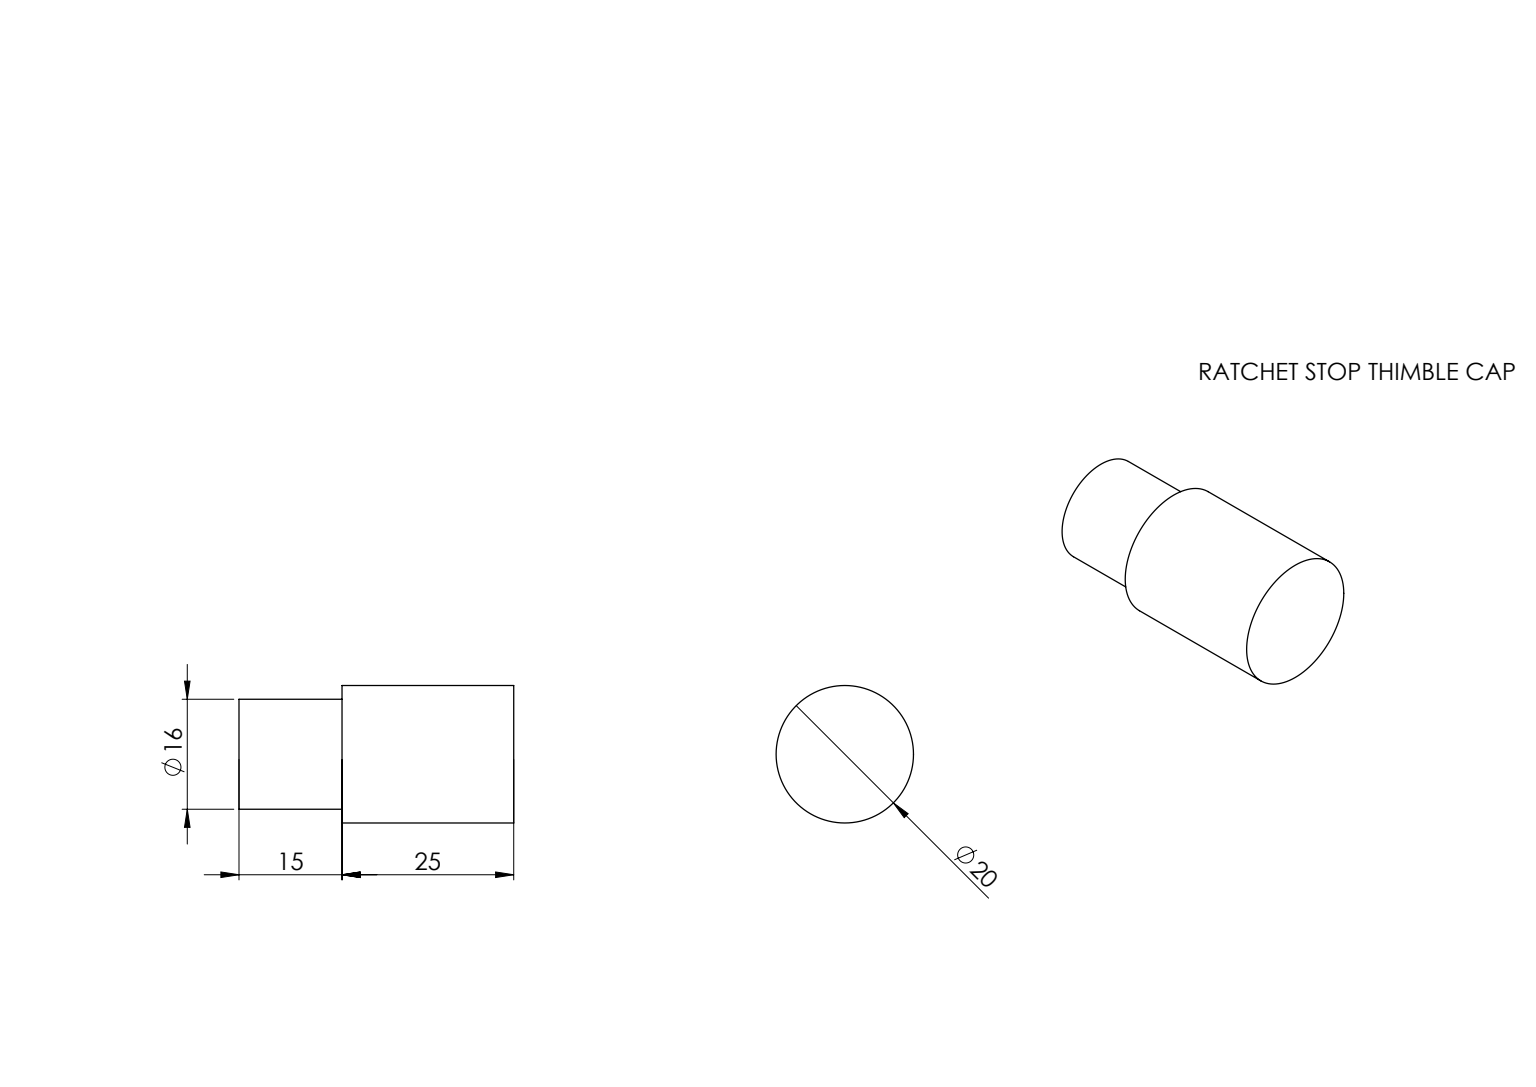
ISO-10303-21;
HEADER;
FILE_DESCRIPTION (('STEP AP214'),
    '1' );
FILE_NAME ('Ratchet Stop Thimble Cap.step',
    '2026-10-22T12:35:56',
    ( '' ),
    ( '' ),
    'SwSTEP 2.0',
    'SolidWorks 2026',
    '' );
FILE_SCHEMA (( 'AUTOMOTIVE_DESIGN' ));
ENDSEC;

DATA;
#21=PRESENTATION_STYLE_ASSIGNMENT (( #2824 ) ) ;
#28=EDGE_CURVE ( 'NONE', #1232, #2394, #2025, .T. ) ;
#41=CARTESIAN_POINT ( 'NONE',  ( 155.0000000000000284, -6.316519372592878167E-15, 2.499999999999999556 ) ) ;
#44=EDGE_CURVE ( 'NONE', #1232, #2037, #954, .T. ) ;
#58=VECTOR ( 'NONE', #2842, 1000.000000000000000 ) ;
#61=CLOSED_SHELL ( 'NONE', ( #1282, #587, #178, #1971, #3042, #967, #2402, #1991, #3073, #2520 ) ) ;
#68=CARTESIAN_POINT ( 'NONE',  ( 180.0000000000000284, -6.928842772166554697E-15, 7.500000000000000000 ) ) ;
#78=CARTESIAN_POINT ( 'NONE',  ( 180.0000000000000284, -6.928842772166554697E-15, 7.500000000000000000 ) ) ;
#80=DIRECTION ( 'NONE',  ( 1.000000000000000000, 0.000000000000000000, 0.000000000000000000 ) ) ;
#90=DIRECTION ( 'NONE',  ( -1.000000000000000000, -0.000000000000000000, -0.000000000000000000 ) ) ;
#91=VERTEX_POINT ( 'NONE', #398 ) ;
#94=SHAPE_DEFINITION_REPRESENTATION ( #2508, #2591 ) ;
#130=FACE_OUTER_BOUND ( 'NONE', #879, .T. ) ;
#132=CARTESIAN_POINT ( 'NONE',  ( 155.0000000000000284, -5.949125332848671934E-15, -0.5000000000000004441 ) ) ;
#142=ORIENTED_EDGE ( 'NONE', *, *, #1580, .F. ) ;
#150=CARTESIAN_POINT ( 'NONE',  ( 140.0000000000000000, -6.928842772166554697E-15, 15.50000000000000000 ) ) ;
#166=CARTESIAN_POINT ( 'NONE',  ( 140.0000000000000000, -6.928842772166554697E-15, 7.500000000000000000 ) ) ;
#178=ADVANCED_FACE ( 'NONE', ( #1464 ), #509, .T. ) ;
#189=( LENGTH_UNIT ( ) NAMED_UNIT ( * ) SI_UNIT ( .MILLI., .METRE. ) );
#194=CARTESIAN_POINT ( 'NONE',  ( 155.0000000000000284, -6.928842772166554697E-15, 7.500000000000000000 ) ) ;
#195=CIRCLE ( 'NONE', #1445, 10.00000000000000178 ) ;
#208=DIRECTION ( 'NONE',  ( 0.000000000000000000, 0.000000000000000000, 1.000000000000000000 ) ) ;
#212=CARTESIAN_POINT ( 'NONE',  ( 180.0000000000000284, -5.704195973019200848E-15, -2.500000000000002220 ) ) ;
#228=DIRECTION ( 'NONE',  ( 1.000000000000000000, 0.000000000000000000, 0.000000000000000000 ) ) ;
#245=ORIENTED_EDGE ( 'NONE', *, *, #981, .F. ) ;
#252=EDGE_CURVE ( 'NONE', #466, #91, #1941, .T. ) ;
#263=AXIS2_PLACEMENT_3D ( 'NONE', #1782, #798, #1552 ) ;
#286=CARTESIAN_POINT ( 'NONE',  ( 140.0000000000000000, -6.316519372592878167E-15, 2.499999999999999556 ) ) ;
#290=PRODUCT_DEFINITION_CONTEXT ( 'detailed design', #3029, 'design' ) ;
#298=EDGE_CURVE ( 'NONE', #3130, #2427, #2917, .T. ) ;
#304=CARTESIAN_POINT ( 'NONE',  ( 180.0000000000000284, -6.928842772166554697E-15, 7.500000000000000000 ) ) ;
#309=( NAMED_UNIT ( * ) SI_UNIT ( $, .STERADIAN. ) SOLID_ANGLE_UNIT ( ) );
#332=ORIENTED_EDGE ( 'NONE', *, *, #28, .F. ) ;
#338=FACE_OUTER_BOUND ( 'NONE', #1623, .T. ) ;
#339=AXIS2_PLACEMENT_3D ( 'NONE', #2130, #2093, #2543 ) ;
#347=CARTESIAN_POINT ( 'NONE',  ( 180.0000000000000284, -6.928842772166554697E-15, 17.50000000000000000 ) ) ;
#368=CARTESIAN_POINT ( 'NONE',  ( 140.0000000000000000, -6.928842772166554697E-15, 7.500000000000000000 ) ) ;
#395=AXIS2_PLACEMENT_3D ( 'NONE', #2044, #2788, #565 ) ;
#396=MECHANICAL_DESIGN_GEOMETRIC_PRESENTATION_REPRESENTATION('',(#2111),#1957);
#398=CARTESIAN_POINT ( 'NONE',  ( 155.0000000000000284, -6.928842772166554697E-15, 17.50000000000000000 ) ) ;
#407=DIRECTION ( 'NONE',  ( 0.000000000000000000, 0.000000000000000000, -1.000000000000000000 ) ) ;
#412=ORIENTED_EDGE ( 'NONE', *, *, #843, .T. ) ;
#418=PLANE ( 'NONE',  #2778 ) ;
#430=ORIENTED_EDGE ( 'NONE', *, *, #981, .T. ) ;
#433=DIRECTION ( 'NONE',  ( 1.000000000000000000, 0.000000000000000000, 0.000000000000000000 ) ) ;
#466=VERTEX_POINT ( 'NONE', #347 ) ;
#473=AXIS2_PLACEMENT_3D ( 'NONE', #1752, #228, #2224 ) ;
#479=VERTEX_POINT ( 'NONE', #286 ) ;
#498=ORIENTED_EDGE ( 'NONE', *, *, #1931, .T. ) ;
#509=CYLINDRICAL_SURFACE ( 'NONE', #747, 8.000000000000000000 ) ;
#554=DIRECTION ( 'NONE',  ( -1.000000000000000000, -0.000000000000000000, -0.000000000000000000 ) ) ;
#557=( LENGTH_UNIT ( ) NAMED_UNIT ( * ) SI_UNIT ( .MILLI., .METRE. ) );
#565=DIRECTION ( 'NONE',  ( 0.000000000000000000, 0.000000000000000000, 1.000000000000000000 ) ) ;
#583=CYLINDRICAL_SURFACE ( 'NONE', #2281, 10.00000000000000178 ) ;
#584=( NAMED_UNIT ( * ) PLANE_ANGLE_UNIT ( ) SI_UNIT ( $, .RADIAN. ) );
#587=ADVANCED_FACE ( 'NONE', ( #1804 ), #785, .F. ) ;
#597=CARTESIAN_POINT ( 'NONE',  ( 155.0000000000000284, -5.704195973019200848E-15, -2.500000000000002220 ) ) ;
#617=ORIENTED_EDGE ( 'NONE', *, *, #252, .T. ) ;
#633=( GEOMETRIC_REPRESENTATION_CONTEXT ( 3 ) GLOBAL_UNCERTAINTY_ASSIGNED_CONTEXT ( ( #2364 ) ) GLOBAL_UNIT_ASSIGNED_CONTEXT ( ( #189, #684, #1683 ) ) REPRESENTATION_CONTEXT ( 'NONE', 'WORKASPACE' ) );
#643=ORIENTED_EDGE ( 'NONE', *, *, #44, .T. ) ;
#644=DIRECTION ( 'NONE',  ( 0.000000000000000000, 0.000000000000000000, -1.000000000000000000 ) ) ;
#646=PLANE ( 'NONE',  #339 ) ;
#653=FACE_OUTER_BOUND ( 'NONE', #990, .T. ) ;
#663=ORIENTED_EDGE ( 'NONE', *, *, #843, .F. ) ;
#666=CARTESIAN_POINT ( 'NONE',  ( 155.0000000000000284, -6.928842772166554697E-15, 7.500000000000000000 ) ) ;
#672=CARTESIAN_POINT ( 'NONE',  ( 155.0000000000000284, -6.928842772166554697E-15, 7.500000000000000000 ) ) ;
#675=ORIENTED_EDGE ( 'NONE', *, *, #1886, .F. ) ;
#684=( NAMED_UNIT ( * ) PLANE_ANGLE_UNIT ( ) SI_UNIT ( $, .RADIAN. ) );
#712=DIRECTION ( 'NONE',  ( 1.000000000000000000, 0.000000000000000000, 0.000000000000000000 ) ) ;
#737=ORIENTED_EDGE ( 'NONE', *, *, #1525, .T. ) ;
#747=AXIS2_PLACEMENT_3D ( 'NONE', #194, #1501, #208 ) ;
#785=CYLINDRICAL_SURFACE ( 'NONE', #395, 5.000000000000000888 ) ;
#794=ORIENTED_EDGE ( 'NONE', *, *, #28, .T. ) ;
#798=DIRECTION ( 'NONE',  ( 1.000000000000000000, 0.000000000000000000, 0.000000000000000000 ) ) ;
#800=CARTESIAN_POINT ( 'NONE',  ( 155.0000000000000284, -6.928842772166554697E-15, 12.50000000000000000 ) ) ;
#843=EDGE_CURVE ( 'NONE', #2350, #2807, #1836, .T. ) ;
#863=CARTESIAN_POINT ( 'NONE',  ( 140.0000000000000000, -6.928842772166554697E-15, 12.50000000000000000 ) ) ;
#865=DIRECTION ( 'NONE',  ( 0.000000000000000000, 0.000000000000000000, 1.000000000000000000 ) ) ;
#873=UNCERTAINTY_MEASURE_WITH_UNIT (LENGTH_MEASURE( 1.000000000000000082E-05 ), #3007, 'distance_accuracy_value', 'NONE');
#878=CARTESIAN_POINT ( 'NONE',  ( 155.0000000000000284, -6.928842772166554697E-15, 7.500000000000000000 ) ) ;
#879=EDGE_LOOP ( 'NONE', ( #2061, #2408 ) ) ;
#903=PRODUCT_CONTEXT ( 'NONE', #969, 'mechanical' ) ;
#940=CARTESIAN_POINT ( 'NONE',  ( 180.0000000000000284, -5.704195973019200848E-15, -2.500000000000002220 ) ) ;
#954=CIRCLE ( 'NONE', #1215, 5.000000000000000000 ) ;
#955=DIRECTION ( 'NONE',  ( -1.000000000000000000, -0.000000000000000000, -0.000000000000000000 ) ) ;
#958=CARTESIAN_POINT ( 'NONE',  ( 180.0000000000000284, -6.928842772166554697E-15, 17.50000000000000000 ) ) ;
#963=FACE_OUTER_BOUND ( 'NONE', #1238, .T. ) ;
#967=ADVANCED_FACE ( 'NONE', ( #2453 ), #2960, .F. ) ;
#969=APPLICATION_CONTEXT ( 'automotive_design' ) ;
#981=EDGE_CURVE ( 'NONE', #2037, #479, #1478, .T. ) ;
#985=AXIS2_PLACEMENT_3D ( 'NONE', #1976, #2688, #2443 ) ;
#990=EDGE_LOOP ( 'NONE', ( #2913, #1504 ) ) ;
#1000=AXIS2_PLACEMENT_3D ( 'NONE', #672, #1412, #2437 ) ;
#1003=VECTOR ( 'NONE', #1553, 1000.000000000000000 ) ;
#1006=EDGE_CURVE ( 'NONE', #2037, #1232, #2098, .T. ) ;
#1017=( NAMED_UNIT ( * ) SI_UNIT ( $, .STERADIAN. ) SOLID_ANGLE_UNIT ( ) );
#1095=ORIENTED_EDGE ( 'NONE', *, *, #2970, .F. ) ;
#1111=CIRCLE ( 'NONE', #1320, 10.00000000000000178 ) ;
#1129=DIRECTION ( 'NONE',  ( 1.000000000000000000, 0.000000000000000000, 0.000000000000000000 ) ) ;
#1139=ADVANCED_BREP_SHAPE_REPRESENTATION ( '', ( #2105, #2878 ), #1375 ) ;
#1152=EDGE_LOOP ( 'NONE', ( #2145, #412, #1160, #2143 ) ) ;
#1160=ORIENTED_EDGE ( 'NONE', *, *, #2742, .T. ) ;
#1161=AXIS2_PLACEMENT_3D ( 'NONE', #1671, #2404, #2221 ) ;
#1207=ORIENTED_EDGE ( 'NONE', *, *, #2422, .T. ) ;
#1215=AXIS2_PLACEMENT_3D ( 'NONE', #1827, #1332, #1802 ) ;
#1219=CIRCLE ( 'NONE', #2885, 8.000000000000000000 ) ;
#1232=VERTEX_POINT ( 'NONE', #2371 ) ;
#1238=EDGE_LOOP ( 'NONE', ( #1589, #1095 ) ) ;
#1264=PRODUCT_DEFINITION ( 'UNKNOWN', '', #1910, #290 ) ;
#1265=AXIS2_PLACEMENT_3D ( 'NONE', #368, #80, #3066 ) ;
#1270=AXIS2_PLACEMENT_3D ( 'NONE', #78, #1129, #644 ) ;
#1282=ADVANCED_FACE ( 'NONE', ( #2116 ), #583, .T. ) ;
#1284=CARTESIAN_POINT ( 'NONE',  ( 140.0000000000000000, -6.928842772166554697E-15, 7.500000000000000000 ) ) ;
#1299=DIRECTION ( 'NONE',  ( 1.000000000000000000, 0.000000000000000000, 0.000000000000000000 ) ) ;
#1300=CIRCLE ( 'NONE', #263, 8.000000000000000000 ) ;
#1319=ORIENTED_EDGE ( 'NONE', *, *, #298, .F. ) ;
#1320=AXIS2_PLACEMENT_3D ( 'NONE', #878, #2334, #1388 ) ;
#1323=DIRECTION ( 'NONE',  ( 0.000000000000000000, 0.000000000000000000, 1.000000000000000000 ) ) ;
#1332=DIRECTION ( 'NONE',  ( 1.000000000000000000, 0.000000000000000000, 0.000000000000000000 ) ) ;
#1337=VECTOR ( 'NONE', #554, 1000.000000000000000 ) ;
#1342=VERTEX_POINT ( 'NONE', #150 ) ;
#1352=ORIENTED_EDGE ( 'NONE', *, *, #44, .F. ) ;
#1375=( GEOMETRIC_REPRESENTATION_CONTEXT ( 3 ) GLOBAL_UNCERTAINTY_ASSIGNED_CONTEXT ( ( #1894 ) ) GLOBAL_UNIT_ASSIGNED_CONTEXT ( ( #557, #584, #1017 ) ) REPRESENTATION_CONTEXT ( 'NONE', 'WORKASPACE' ) );
#1388=DIRECTION ( 'NONE',  ( 0.000000000000000000, 0.000000000000000000, -1.000000000000000000 ) ) ;
#1412=DIRECTION ( 'NONE',  ( -1.000000000000000000, -0.000000000000000000, -0.000000000000000000 ) ) ;
#1419=EDGE_LOOP ( 'NONE', ( #142, #1925, #1642, #1594 ) ) ;
#1431=CARTESIAN_POINT ( 'NONE',  ( 155.0000000000000284, -6.316519372592878167E-15, 2.499999999999999556 ) ) ;
#1445=AXIS2_PLACEMENT_3D ( 'NONE', #304, #2774, #2511 ) ;
#1454=FACE_BOUND ( 'NONE', #2335, .T. ) ;
#1459=AXIS2_PLACEMENT_3D ( 'NONE', #1800, #2389, #1891 ) ;
#1464=FACE_OUTER_BOUND ( 'NONE', #1152, .T. ) ;
#1472=CARTESIAN_POINT ( 'NONE',  ( 155.0000000000000284, -6.928842772166554697E-15, 15.50000000000000000 ) ) ;
#1478=LINE ( 'NONE', #1431, #3191 ) ;
#1492=CARTESIAN_POINT ( 'NONE',  ( 140.0000000000000000, -5.949125332848671934E-15, -0.5000000000000004441 ) ) ;
#1501=DIRECTION ( 'NONE',  ( -1.000000000000000000, -0.000000000000000000, -0.000000000000000000 ) ) ;
#1504=ORIENTED_EDGE ( 'NONE', *, *, #2742, .F. ) ;
#1525=EDGE_CURVE ( 'NONE', #1604, #1342, #2031, .T. ) ;
#1527=SURFACE_SIDE_STYLE ('',( #1547 ) ) ;
#1547=SURFACE_STYLE_FILL_AREA ( #2279 ) ;
#1552=DIRECTION ( 'NONE',  ( 0.000000000000000000, 0.000000000000000000, -1.000000000000000000 ) ) ;
#1553=DIRECTION ( 'NONE',  ( -1.000000000000000000, -0.000000000000000000, -0.000000000000000000 ) ) ;
#1571=CIRCLE ( 'NONE', #2302, 10.00000000000000178 ) ;
#1580=EDGE_CURVE ( 'NONE', #3130, #466, #195, .T. ) ;
#1589=ORIENTED_EDGE ( 'NONE', *, *, #1869, .F. ) ;
#1594=ORIENTED_EDGE ( 'NONE', *, *, #252, .F. ) ;
#1604=VERTEX_POINT ( 'NONE', #1472 ) ;
#1617=ORIENTED_EDGE ( 'NONE', *, *, #2613, .T. ) ;
#1618=CIRCLE ( 'NONE', #985, 8.000000000000000000 ) ;
#1622=CYLINDRICAL_SURFACE ( 'NONE', #2464, 8.000000000000000000 ) ;
#1623=EDGE_LOOP ( 'NONE', ( #1352, #1652 ) ) ;
#1637=ORIENTED_EDGE ( 'NONE', *, *, #2639, .F. ) ;
#1642=ORIENTED_EDGE ( 'NONE', *, *, #2970, .T. ) ;
#1648=DIRECTION ( 'NONE',  ( 1.000000000000000000, 0.000000000000000000, 0.000000000000000000 ) ) ;
#1652=ORIENTED_EDGE ( 'NONE', *, *, #1006, .F. ) ;
#1671=CARTESIAN_POINT ( 'NONE',  ( 155.0000000000000284, -6.928842772166554697E-15, 7.500000000000000000 ) ) ;
#1683=( NAMED_UNIT ( * ) SI_UNIT ( $, .STERADIAN. ) SOLID_ANGLE_UNIT ( ) );
#1696=CARTESIAN_POINT ( 'NONE',  ( 140.0000000000000000, -6.928842772166554697E-15, 7.500000000000000000 ) ) ;
#1711=EDGE_LOOP ( 'NONE', ( #643, #430, #2950, #332 ) ) ;
#1748=VECTOR ( 'NONE', #1750, 1000.000000000000000 ) ;
#1749=EDGE_LOOP ( 'NONE', ( #663, #675, #737, #1763 ) ) ;
#1750=DIRECTION ( 'NONE',  ( -1.000000000000000000, -0.000000000000000000, -0.000000000000000000 ) ) ;
#1752=CARTESIAN_POINT ( 'NONE',  ( 155.0000000000000284, -6.928842772166554697E-15, 7.500000000000000000 ) ) ;
#1763=ORIENTED_EDGE ( 'NONE', *, *, #2556, .T. ) ;
#1782=CARTESIAN_POINT ( 'NONE',  ( 155.0000000000000284, -6.928842772166554697E-15, 7.500000000000000000 ) ) ;
#1800=CARTESIAN_POINT ( 'NONE',  ( 180.0000000000000284, -6.928842772166554697E-15, 7.500000000000000000 ) ) ;
#1802=DIRECTION ( 'NONE',  ( 0.000000000000000000, 0.000000000000000000, -1.000000000000000000 ) ) ;
#1804=FACE_OUTER_BOUND ( 'NONE', #1711, .T. ) ;
#1827=CARTESIAN_POINT ( 'NONE',  ( 155.0000000000000284, -6.928842772166554697E-15, 7.500000000000000000 ) ) ;
#1831=FACE_OUTER_BOUND ( 'NONE', #1749, .T. ) ;
#1836=LINE ( 'NONE', #2100, #58 ) ;
#1837=DIRECTION ( 'NONE',  ( 1.000000000000000000, 0.000000000000000000, 0.000000000000000000 ) ) ;
#1869=EDGE_CURVE ( 'NONE', #91, #2427, #1878, .T. ) ;
#1878=CIRCLE ( 'NONE', #473, 10.00000000000000178 ) ;
#1886=EDGE_CURVE ( 'NONE', #1604, #2350, #1618, .T. ) ;
#1891=DIRECTION ( 'NONE',  ( 0.000000000000000000, 0.000000000000000000, 1.000000000000000000 ) ) ;
#1894=UNCERTAINTY_MEASURE_WITH_UNIT (LENGTH_MEASURE( 1.000000000000000082E-05 ), #557, 'distance_accuracy_value', 'NONE');
#1910=PRODUCT_DEFINITION_FORMATION_WITH_SPECIFIED_SOURCE ( 'ANY', '', #2771, .NOT_KNOWN. ) ;
#1919=DIRECTION ( 'NONE',  ( 0.000000000000000000, 0.000000000000000000, -1.000000000000000000 ) ) ;
#1925=ORIENTED_EDGE ( 'NONE', *, *, #298, .T. ) ;
#1931=EDGE_CURVE ( 'NONE', #2350, #1604, #1300, .T. ) ;
#1935=DIRECTION ( 'NONE',  ( 0.000000000000000000, 0.000000000000000000, -1.000000000000000000 ) ) ;
#1941=LINE ( 'NONE', #958, #1951 ) ;
#1951=VECTOR ( 'NONE', #2702, 1000.000000000000000 ) ;
#1957=( GEOMETRIC_REPRESENTATION_CONTEXT ( 3 ) GLOBAL_UNCERTAINTY_ASSIGNED_CONTEXT ( ( #873 ) ) GLOBAL_UNIT_ASSIGNED_CONTEXT ( ( #3007, #3022, #309 ) ) REPRESENTATION_CONTEXT ( 'NONE', 'WORKASPACE' ) );
#1965=DIRECTION ( 'NONE',  ( 1.000000000000000000, 0.000000000000000000, 0.000000000000000000 ) ) ;
#1971=ADVANCED_FACE ( 'NONE', ( #653, #2135 ), #3028, .F. ) ;
#1976=CARTESIAN_POINT ( 'NONE',  ( 155.0000000000000284, -6.928842772166554697E-15, 7.500000000000000000 ) ) ;
#1991=ADVANCED_FACE ( 'NONE', ( #2592 ), #2120, .T. ) ;
#2011=ORIENTED_EDGE ( 'NONE', *, *, #2422, .F. ) ;
#2025=LINE ( 'NONE', #800, #1003 ) ;
#2031=LINE ( 'NONE', #2480, #1337 ) ;
#2037=VERTEX_POINT ( 'NONE', #41 ) ;
#2042=AXIS2_PLACEMENT_3D ( 'NONE', #166, #2182, #2956 ) ;
#2044=CARTESIAN_POINT ( 'NONE',  ( 155.0000000000000284, -6.928842772166554697E-15, 7.500000000000000000 ) ) ;
#2061=ORIENTED_EDGE ( 'NONE', *, *, #2639, .T. ) ;
#2093=DIRECTION ( 'NONE',  ( 1.000000000000000000, 0.000000000000000000, 0.000000000000000000 ) ) ;
#2098=CIRCLE ( 'NONE', #1161, 5.000000000000000000 ) ;
#2100=CARTESIAN_POINT ( 'NONE',  ( 155.0000000000000284, -5.949125332848671934E-15, -0.5000000000000004441 ) ) ;
#2105=MANIFOLD_SOLID_BREP ( 'Boss-Extrude1', #61 ) ;
#2111=STYLED_ITEM ( 'NONE', ( #21 ), #1139 ) ;
#2116=FACE_OUTER_BOUND ( 'NONE', #1419, .T. ) ;
#2120=CYLINDRICAL_SURFACE ( 'NONE', #1459, 10.00000000000000178 ) ;
#2130=CARTESIAN_POINT ( 'NONE',  ( 155.0000000000000284, -6.928842772166554697E-15, 7.500000000000000000 ) ) ;
#2135=FACE_BOUND ( 'NONE', #2178, .T. ) ;
#2143=ORIENTED_EDGE ( 'NONE', *, *, #1525, .F. ) ;
#2145=ORIENTED_EDGE ( 'NONE', *, *, #1931, .F. ) ;
#2150=AXIS2_PLACEMENT_3D ( 'NONE', #2627, #1648, #1919 ) ;
#2178=EDGE_LOOP ( 'NONE', ( #1617, #1207 ) ) ;
#2182=DIRECTION ( 'NONE',  ( 1.000000000000000000, 0.000000000000000000, 0.000000000000000000 ) ) ;
#2197=AXIS2_PLACEMENT_3D ( 'NONE', #1284, #1299, #407 ) ;
#2221=DIRECTION ( 'NONE',  ( 0.000000000000000000, 0.000000000000000000, -1.000000000000000000 ) ) ;
#2224=DIRECTION ( 'NONE',  ( 0.000000000000000000, 0.000000000000000000, -1.000000000000000000 ) ) ;
#2238=EDGE_LOOP ( 'NONE', ( #245, #2922, #794, #2011 ) ) ;
#2250=STYLED_ITEM('',(#3271),#2105);
#2279=FILL_AREA_STYLE ('',( #2545 ) ) ;
#2281=AXIS2_PLACEMENT_3D ( 'NONE', #68, #3099, #865 ) ;
#2302=AXIS2_PLACEMENT_3D ( 'NONE', #2657, #433, #2414 ) ;
#2334=DIRECTION ( 'NONE',  ( 1.000000000000000000, 0.000000000000000000, 0.000000000000000000 ) ) ;
#2335=EDGE_LOOP ( 'NONE', ( #2354, #498 ) ) ;
#2350=VERTEX_POINT ( 'NONE', #132 ) ;
#2354=ORIENTED_EDGE ( 'NONE', *, *, #1886, .T. ) ;
#2364=UNCERTAINTY_MEASURE_WITH_UNIT (LENGTH_MEASURE( 1.000000000000000082E-05 ), #189, 'distance_accuracy_value', 'NONE');
#2371=CARTESIAN_POINT ( 'NONE',  ( 155.0000000000000284, -6.928842772166554697E-15, 12.50000000000000000 ) ) ;
#2389=DIRECTION ( 'NONE',  ( -1.000000000000000000, -0.000000000000000000, -0.000000000000000000 ) ) ;
#2394=VERTEX_POINT ( 'NONE', #863 ) ;
#2402=ADVANCED_FACE ( 'NONE', ( #338 ), #646, .F. ) ;
#2404=DIRECTION ( 'NONE',  ( 1.000000000000000000, 0.000000000000000000, 0.000000000000000000 ) ) ;
#2408=ORIENTED_EDGE ( 'NONE', *, *, #1580, .T. ) ;
#2414=DIRECTION ( 'NONE',  ( 0.000000000000000000, 0.000000000000000000, -1.000000000000000000 ) ) ;
#2422=EDGE_CURVE ( 'NONE', #479, #2394, #2513, .T. ) ;
#2427=VERTEX_POINT ( 'NONE', #597 ) ;
#2437=DIRECTION ( 'NONE',  ( 0.000000000000000000, 0.000000000000000000, 1.000000000000000000 ) ) ;
#2443=DIRECTION ( 'NONE',  ( 0.000000000000000000, 0.000000000000000000, -1.000000000000000000 ) ) ;
#2453=FACE_OUTER_BOUND ( 'NONE', #2238, .T. ) ;
#2454=CIRCLE ( 'NONE', #2042, 8.000000000000000000 ) ;
#2464=AXIS2_PLACEMENT_3D ( 'NONE', #2820, #90, #1323 ) ;
#2480=CARTESIAN_POINT ( 'NONE',  ( 155.0000000000000284, -6.928842772166554697E-15, 15.50000000000000000 ) ) ;
#2508=PRODUCT_DEFINITION_SHAPE ( 'NONE', 'NONE',  #1264 ) ;
#2511=DIRECTION ( 'NONE',  ( 0.000000000000000000, 0.000000000000000000, -1.000000000000000000 ) ) ;
#2513=CIRCLE ( 'NONE', #1265, 5.000000000000000000 ) ;
#2516=SHAPE_REPRESENTATION_RELATIONSHIP ( 'NONE' , 'NONE' ,  #2591, #1139 ) ;
#2520=ADVANCED_FACE ( 'NONE', ( #1454, #963 ), #418, .F. ) ;
#2543=DIRECTION ( 'NONE',  ( 0.000000000000000000, 0.000000000000000000, -1.000000000000000000 ) ) ;
#2545=FILL_AREA_STYLE_COLOUR ( '', #2733 ) ;
#2556=EDGE_CURVE ( 'NONE', #1342, #2807, #1219, .T. ) ;
#2582=EDGE_LOOP ( 'NONE', ( #1319, #1637, #617, #2939 ) ) ;
#2591=SHAPE_REPRESENTATION ( 'Ratchet Stop Thimble Cap', ( #2878 ), #1375 ) ;
#2592=FACE_OUTER_BOUND ( 'NONE', #2582, .T. ) ;
#2613=EDGE_CURVE ( 'NONE', #2394, #479, #2712, .T. ) ;
#2627=CARTESIAN_POINT ( 'NONE',  ( 140.0000000000000000, -6.928842772166554697E-15, 7.500000000000000000 ) ) ;
#2639=EDGE_CURVE ( 'NONE', #466, #3130, #1571, .T. ) ;
#2643=DIRECTION ( 'NONE',  ( 0.000000000000000000, 0.000000000000000000, -1.000000000000000000 ) ) ;
#2657=CARTESIAN_POINT ( 'NONE',  ( 180.0000000000000284, -6.928842772166554697E-15, 7.500000000000000000 ) ) ;
#2688=DIRECTION ( 'NONE',  ( 1.000000000000000000, 0.000000000000000000, 0.000000000000000000 ) ) ;
#2702=DIRECTION ( 'NONE',  ( -1.000000000000000000, -0.000000000000000000, -0.000000000000000000 ) ) ;
#2712=CIRCLE ( 'NONE', #2150, 5.000000000000000000 ) ;
#2733=COLOUR_RGB ( '',0.8941176470588234615, 0.8941176470588234615, 0.8941176470588234615 ) ;
#2742=EDGE_CURVE ( 'NONE', #2807, #1342, #2454, .T. ) ;
#2771=PRODUCT ( 'Ratchet Stop Thimble Cap', 'Ratchet Stop Thimble Cap', '', ( #903 ) ) ;
#2774=DIRECTION ( 'NONE',  ( 1.000000000000000000, 0.000000000000000000, 0.000000000000000000 ) ) ;
#2778=AXIS2_PLACEMENT_3D ( 'NONE', #666, #1965, #1935 ) ;
#2788=DIRECTION ( 'NONE',  ( -1.000000000000000000, -0.000000000000000000, -0.000000000000000000 ) ) ;
#2799=DIRECTION ( 'NONE',  ( 0.000000000000000000, 0.000000000000000000, 1.000000000000000000 ) ) ;
#2807=VERTEX_POINT ( 'NONE', #1492 ) ;
#2820=CARTESIAN_POINT ( 'NONE',  ( 155.0000000000000284, -6.928842772166554697E-15, 7.500000000000000000 ) ) ;
#2824=SURFACE_STYLE_USAGE ( .BOTH. , #1527 ) ;
#2842=DIRECTION ( 'NONE',  ( -1.000000000000000000, -0.000000000000000000, -0.000000000000000000 ) ) ;
#2878=AXIS2_PLACEMENT_3D ( 'NONE', #3071, #2799, #1837 ) ;
#2885=AXIS2_PLACEMENT_3D ( 'NONE', #1696, #712, #2643 ) ;
#2913=ORIENTED_EDGE ( 'NONE', *, *, #2556, .F. ) ;
#2917=LINE ( 'NONE', #940, #1748 ) ;
#2922=ORIENTED_EDGE ( 'NONE', *, *, #1006, .T. ) ;
#2939=ORIENTED_EDGE ( 'NONE', *, *, #1869, .T. ) ;
#2950=ORIENTED_EDGE ( 'NONE', *, *, #2613, .F. ) ;
#2956=DIRECTION ( 'NONE',  ( 0.000000000000000000, 0.000000000000000000, -1.000000000000000000 ) ) ;
#2960=CYLINDRICAL_SURFACE ( 'NONE', #1000, 5.000000000000000888 ) ;
#2970=EDGE_CURVE ( 'NONE', #2427, #91, #1111, .T. ) ;
#3007=( LENGTH_UNIT ( ) NAMED_UNIT ( * ) SI_UNIT ( .MILLI., .METRE. ) );
#3022=( NAMED_UNIT ( * ) PLANE_ANGLE_UNIT ( ) SI_UNIT ( $, .RADIAN. ) );
#3028=PLANE ( 'NONE',  #2197 ) ;
#3029=APPLICATION_CONTEXT ( 'automotive_design' ) ;
#3042=ADVANCED_FACE ( 'NONE', ( #1831 ), #1622, .T. ) ;
#3066=DIRECTION ( 'NONE',  ( 0.000000000000000000, 0.000000000000000000, -1.000000000000000000 ) ) ;
#3071=CARTESIAN_POINT ( 'NONE',  ( 0.000000000000000000, 0.000000000000000000, 0.000000000000000000 ) ) ;
#3073=ADVANCED_FACE ( 'NONE', ( #130 ), #3077, .T. ) ;
#3077=PLANE ( 'NONE',  #1270 ) ;
#3099=DIRECTION ( 'NONE',  ( -1.000000000000000000, -0.000000000000000000, -0.000000000000000000 ) ) ;
#3123=MECHANICAL_DESIGN_GEOMETRIC_PRESENTATION_REPRESENTATION('',(#2250),#633);
#3130=VERTEX_POINT ( 'NONE', #212 ) ;
#3191=VECTOR ( 'NONE', #955, 1000.000000000000000 ) ;
#3265=COLOUR_RGB('Off White',0.89,0.88,0.83);
#3266=FILL_AREA_STYLE_COLOUR('',#3265);
#3267=FILL_AREA_STYLE('',(#3266));
#3268=SURFACE_STYLE_FILL_AREA(#3267);
#3269=SURFACE_SIDE_STYLE('',(#3268));
#3270=SURFACE_STYLE_USAGE(.BOTH.,#3269);
#3271=PRESENTATION_STYLE_ASSIGNMENT((#3270));
ENDSEC;
END-ISO-10303-21;
